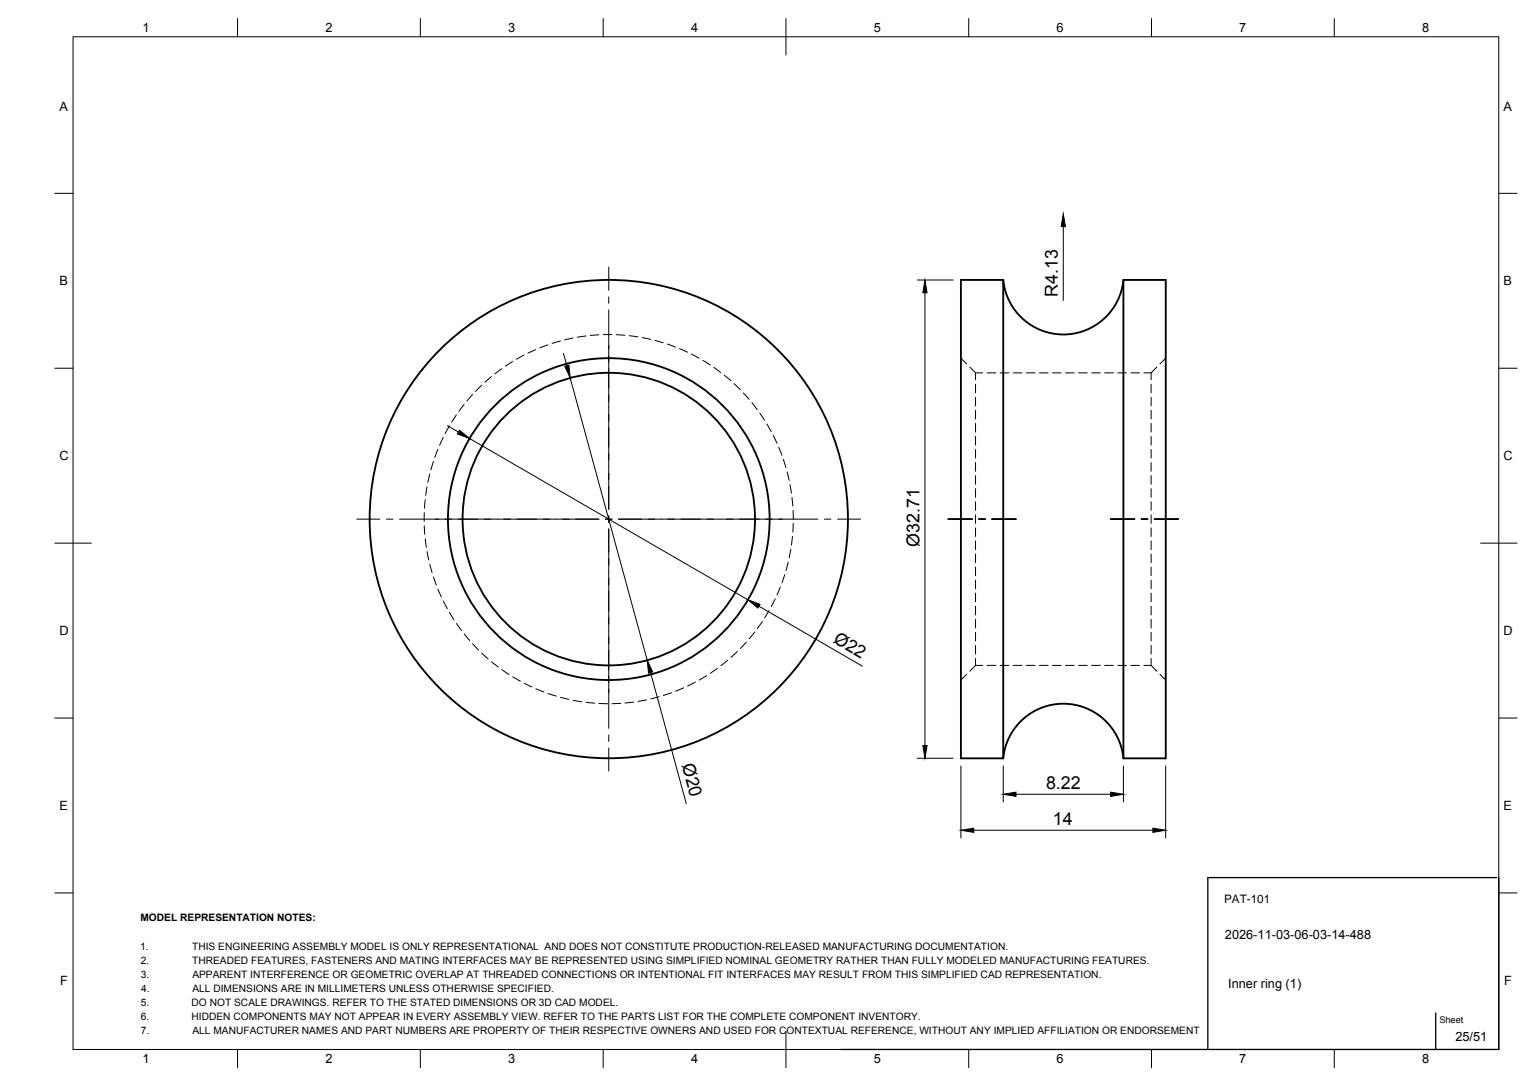
ISO-10303-21;
HEADER;
/* Generated by software containing ST-Developer
 * from STEP Tools, Inc. (www.steptools.com) 
 */

FILE_DESCRIPTION(
/* description */ ('Spur gear reduction stage 2-1 on bearing plates'),
/* implementation_level */ '2;1');

FILE_NAME(
/* name */ 'Inner ring (1).step',
/* time_stamp */ '2026-10-28T03:22:07-07:00',
/* author */ (''),
/* organization */ (''),
/* preprocessor_version */ 'ST-DEVELOPER v20.2',
/* originating_system */ 'Autodesk Translation Framework v15.17.0.0',
/* authorisation */ '');

FILE_SCHEMA (('AUTOMOTIVE_DESIGN { 1 0 10303 214 3 1 1 }'));
ENDSEC;

DATA;
#10=MECHANICAL_DESIGN_GEOMETRIC_PRESENTATION_REPRESENTATION('',(#972),#53909);
#827=TOROIDAL_SURFACE('',#12283,1.675,0.412776);
#844=CONICAL_SURFACE('',#12294,1.05,0.785398163397449);
#845=CONICAL_SURFACE('',#12301,1.05,0.785398163397449);
#879=SHAPE_REPRESENTATION_RELATIONSHIP('SRR','None',#54108,#922);
#922=ADVANCED_BREP_SHAPE_REPRESENTATION('',(#1028),#53882);
#972=STYLED_ITEM('',(#54397),#1028);
#1028=MANIFOLD_SOLID_BREP('Body1',#11298);
#1187=FACE_BOUND('',#2495,.T.);
#1188=FACE_BOUND('',#2498,.T.);
#1330=PLANE('',#12296);
#1331=PLANE('',#12299);
#1715=FACE_OUTER_BOUND('',#2490,.T.);
#1716=FACE_OUTER_BOUND('',#2491,.T.);
#1717=FACE_OUTER_BOUND('',#2492,.T.);
#1718=FACE_OUTER_BOUND('',#2493,.T.);
#1719=FACE_OUTER_BOUND('',#2494,.T.);
#1720=FACE_OUTER_BOUND('',#2496,.T.);
#1721=FACE_OUTER_BOUND('',#2497,.T.);
#1722=FACE_OUTER_BOUND('',#2499,.T.);
#2490=EDGE_LOOP('',(#8206,#8207,#8208,#8209,#8210,#8211));
#2491=EDGE_LOOP('',(#8212,#8213,#8214,#8215,#8216));
#2492=EDGE_LOOP('',(#8217,#8218,#8219,#8220));
#2493=EDGE_LOOP('',(#8221,#8222,#8223,#8224));
#2494=EDGE_LOOP('',(#8225));
#2495=EDGE_LOOP('',(#8226));
#2496=EDGE_LOOP('',(#8227,#8228,#8229,#8230,#8231));
#2497=EDGE_LOOP('',(#8232));
#2498=EDGE_LOOP('',(#8233));
#2499=EDGE_LOOP('',(#8234,#8235,#8236,#8237));
#3153=LINE('',#17238,#3794);
#3154=LINE('',#17244,#3795);
#3155=LINE('',#17248,#3796);
#3156=LINE('',#17254,#3797);
#3157=LINE('',#17259,#3798);
#3794=VECTOR('',#14126,1.63531);
#3795=VECTOR('',#14133,1.);
#3796=VECTOR('',#14138,1.05);
#3797=VECTOR('',#14147,1.63531);
#3798=VECTOR('',#14154,1.05);
#4496=CIRCLE('',#12284,1.63531);
#4497=CIRCLE('',#12285,1.63531);
#4498=CIRCLE('',#12286,0.412776);
#4499=CIRCLE('',#12287,1.63531);
#4500=CIRCLE('',#12288,1.63531);
#4501=CIRCLE('',#12290,1.63531);
#4502=CIRCLE('',#12292,1.);
#4503=CIRCLE('',#12293,1.);
#4504=CIRCLE('',#12295,1.1);
#4505=CIRCLE('',#12298,1.63531);
#4506=CIRCLE('',#12300,1.1);
#5074=VERTEX_POINT('',#17227);
#5075=VERTEX_POINT('',#17228);
#5076=VERTEX_POINT('',#17231);
#5077=VERTEX_POINT('',#17233);
#5078=VERTEX_POINT('',#17237);
#5079=VERTEX_POINT('',#17241);
#5080=VERTEX_POINT('',#17243);
#5081=VERTEX_POINT('',#17247);
#5082=VERTEX_POINT('',#17252);
#5083=VERTEX_POINT('',#17256);
#6245=EDGE_CURVE('',#5074,#5075,#4496,.T.);
#6246=EDGE_CURVE('',#5075,#5074,#4497,.T.);
#6247=EDGE_CURVE('',#5075,#5076,#4498,.T.);
#6248=EDGE_CURVE('',#5077,#5076,#4499,.T.);
#6249=EDGE_CURVE('',#5076,#5077,#4500,.T.);
#6250=EDGE_CURVE('',#5077,#5078,#3153,.T.);
#6251=EDGE_CURVE('',#5078,#5078,#4501,.T.);
#6252=EDGE_CURVE('',#5079,#5079,#4502,.T.);
#6253=EDGE_CURVE('',#5079,#5080,#3154,.T.);
#6254=EDGE_CURVE('',#5080,#5080,#4503,.T.);
#6255=EDGE_CURVE('',#5080,#5081,#3155,.T.);
#6256=EDGE_CURVE('',#5081,#5081,#4504,.T.);
#6257=EDGE_CURVE('',#5082,#5082,#4505,.T.);
#6258=EDGE_CURVE('',#5082,#5074,#3156,.T.);
#6259=EDGE_CURVE('',#5083,#5083,#4506,.T.);
#6260=EDGE_CURVE('',#5083,#5079,#3157,.T.);
#8206=ORIENTED_EDGE('',*,*,#6245,.F.);
#8207=ORIENTED_EDGE('',*,*,#6246,.F.);
#8208=ORIENTED_EDGE('',*,*,#6247,.T.);
#8209=ORIENTED_EDGE('',*,*,#6248,.F.);
#8210=ORIENTED_EDGE('',*,*,#6249,.F.);
#8211=ORIENTED_EDGE('',*,*,#6247,.F.);
#8212=ORIENTED_EDGE('',*,*,#6248,.T.);
#8213=ORIENTED_EDGE('',*,*,#6249,.T.);
#8214=ORIENTED_EDGE('',*,*,#6250,.T.);
#8215=ORIENTED_EDGE('',*,*,#6251,.T.);
#8216=ORIENTED_EDGE('',*,*,#6250,.F.);
#8217=ORIENTED_EDGE('',*,*,#6252,.T.);
#8218=ORIENTED_EDGE('',*,*,#6253,.T.);
#8219=ORIENTED_EDGE('',*,*,#6254,.F.);
#8220=ORIENTED_EDGE('',*,*,#6253,.F.);
#8221=ORIENTED_EDGE('',*,*,#6254,.T.);
#8222=ORIENTED_EDGE('',*,*,#6255,.T.);
#8223=ORIENTED_EDGE('',*,*,#6256,.F.);
#8224=ORIENTED_EDGE('',*,*,#6255,.F.);
#8225=ORIENTED_EDGE('',*,*,#6251,.F.);
#8226=ORIENTED_EDGE('',*,*,#6256,.T.);
#8227=ORIENTED_EDGE('',*,*,#6257,.F.);
#8228=ORIENTED_EDGE('',*,*,#6258,.T.);
#8229=ORIENTED_EDGE('',*,*,#6245,.T.);
#8230=ORIENTED_EDGE('',*,*,#6246,.T.);
#8231=ORIENTED_EDGE('',*,*,#6258,.F.);
#8232=ORIENTED_EDGE('',*,*,#6257,.T.);
#8233=ORIENTED_EDGE('',*,*,#6259,.F.);
#8234=ORIENTED_EDGE('',*,*,#6259,.T.);
#8235=ORIENTED_EDGE('',*,*,#6260,.T.);
#8236=ORIENTED_EDGE('',*,*,#6252,.F.);
#8237=ORIENTED_EDGE('',*,*,#6260,.F.);
#10512=CYLINDRICAL_SURFACE('',#12289,1.63531);
#10513=CYLINDRICAL_SURFACE('',#12291,1.);
#10514=CYLINDRICAL_SURFACE('',#12297,1.63531);
#10835=ADVANCED_FACE('',(#1715),#827,.F.);
#10836=ADVANCED_FACE('',(#1716),#10512,.T.);
#10837=ADVANCED_FACE('',(#1717),#10513,.F.);
#10838=ADVANCED_FACE('',(#1718),#844,.F.);
#10839=ADVANCED_FACE('',(#1719,#1187),#1330,.T.);
#10840=ADVANCED_FACE('',(#1720),#10514,.T.);
#10841=ADVANCED_FACE('',(#1721,#1188),#1331,.T.);
#10842=ADVANCED_FACE('',(#1722),#845,.F.);
#11298=CLOSED_SHELL('',(#10835,#10836,#10837,#10838,#10839,#10840,#10841,
#10842));
#12282=AXIS2_PLACEMENT_3D('',#17225,#14110,#14111);
#12283=AXIS2_PLACEMENT_3D('',#17226,#14112,#14113);
#12284=AXIS2_PLACEMENT_3D('',#17229,#14114,#14115);
#12285=AXIS2_PLACEMENT_3D('',#17230,#14116,#14117);
#12286=AXIS2_PLACEMENT_3D('',#17232,#14118,#14119);
#12287=AXIS2_PLACEMENT_3D('',#17234,#14120,#14121);
#12288=AXIS2_PLACEMENT_3D('',#17235,#14122,#14123);
#12289=AXIS2_PLACEMENT_3D('',#17236,#14124,#14125);
#12290=AXIS2_PLACEMENT_3D('',#17239,#14127,#14128);
#12291=AXIS2_PLACEMENT_3D('',#17240,#14129,#14130);
#12292=AXIS2_PLACEMENT_3D('',#17242,#14131,#14132);
#12293=AXIS2_PLACEMENT_3D('',#17245,#14134,#14135);
#12294=AXIS2_PLACEMENT_3D('',#17246,#14136,#14137);
#12295=AXIS2_PLACEMENT_3D('',#17249,#14139,#14140);
#12296=AXIS2_PLACEMENT_3D('',#17250,#14141,#14142);
#12297=AXIS2_PLACEMENT_3D('',#17251,#14143,#14144);
#12298=AXIS2_PLACEMENT_3D('',#17253,#14145,#14146);
#12299=AXIS2_PLACEMENT_3D('',#17255,#14148,#14149);
#12300=AXIS2_PLACEMENT_3D('',#17257,#14150,#14151);
#12301=AXIS2_PLACEMENT_3D('',#17258,#14152,#14153);
#14110=DIRECTION('axis',(0.,0.,1.));
#14111=DIRECTION('refdir',(1.,0.,0.));
#14112=DIRECTION('center_axis',(0.,-1.,0.));
#14113=DIRECTION('ref_axis',(0.,0.,-1.));
#14114=DIRECTION('center_axis',(0.,-1.,0.));
#14115=DIRECTION('ref_axis',(1.,0.,0.));
#14116=DIRECTION('center_axis',(0.,-1.,0.));
#14117=DIRECTION('ref_axis',(1.,0.,0.));
#14118=DIRECTION('center_axis',(1.,0.,1.22464679914735E-16));
#14119=DIRECTION('ref_axis',(-1.22464679914735E-16,0.,1.));
#14120=DIRECTION('center_axis',(0.,1.,0.));
#14121=DIRECTION('ref_axis',(1.,0.,0.));
#14122=DIRECTION('center_axis',(0.,1.,0.));
#14123=DIRECTION('ref_axis',(1.,0.,0.));
#14124=DIRECTION('center_axis',(0.,-1.,0.));
#14125=DIRECTION('ref_axis',(1.,0.,0.));
#14126=DIRECTION('',(0.,1.,0.));
#14127=DIRECTION('center_axis',(0.,-1.,0.));
#14128=DIRECTION('ref_axis',(1.,0.,0.));
#14129=DIRECTION('center_axis',(0.,-1.,0.));
#14130=DIRECTION('ref_axis',(1.,0.,0.));
#14131=DIRECTION('center_axis',(0.,-1.,0.));
#14132=DIRECTION('ref_axis',(1.,0.,0.));
#14133=DIRECTION('',(0.,1.,0.));
#14134=DIRECTION('center_axis',(0.,-1.,0.));
#14135=DIRECTION('ref_axis',(1.,0.,0.));
#14136=DIRECTION('center_axis',(0.,1.,0.));
#14137=DIRECTION('ref_axis',(1.,0.,0.));
#14138=DIRECTION('',(-0.707106781186548,0.707106781186547,-8.65956056235494E-17));
#14139=DIRECTION('center_axis',(0.,-1.,0.));
#14140=DIRECTION('ref_axis',(1.,0.,0.));
#14141=DIRECTION('center_axis',(0.,1.,0.));
#14142=DIRECTION('ref_axis',(0.,0.,1.));
#14143=DIRECTION('center_axis',(0.,-1.,0.));
#14144=DIRECTION('ref_axis',(1.,0.,0.));
#14145=DIRECTION('center_axis',(0.,-1.,0.));
#14146=DIRECTION('ref_axis',(1.,0.,0.));
#14147=DIRECTION('',(0.,1.,0.));
#14148=DIRECTION('center_axis',(0.,-1.,0.));
#14149=DIRECTION('ref_axis',(0.,0.,-1.));
#14150=DIRECTION('center_axis',(0.,-1.,0.));
#14151=DIRECTION('ref_axis',(1.,0.,0.));
#14152=DIRECTION('center_axis',(0.,-1.,0.));
#14153=DIRECTION('ref_axis',(1.,0.,0.));
#14154=DIRECTION('',(0.707106781186548,0.707106781186547,8.65956056235494E-17));
#17225=CARTESIAN_POINT('',(0.,0.,0.));
#17226=CARTESIAN_POINT('Origin',(0.,0.,0.));
#17227=CARTESIAN_POINT('',(-1.63531,-0.410863395882378,-2.00267715711366E-16));
#17228=CARTESIAN_POINT('',(-2.00267715711366E-16,-0.410863395882378,1.63531));
#17229=CARTESIAN_POINT('Origin',(0.,-0.410863395882378,0.));
#17230=CARTESIAN_POINT('Origin',(0.,-0.410863395882378,0.));
#17231=CARTESIAN_POINT('',(-2.00267715711366E-16,0.410863395882378,1.63531));
#17232=CARTESIAN_POINT('Origin',(-2.05128338857182E-16,0.,1.675));
#17233=CARTESIAN_POINT('',(-1.63531,0.410863395882378,2.00267715711366E-16));
#17234=CARTESIAN_POINT('Origin',(0.,0.410863395882378,0.));
#17235=CARTESIAN_POINT('Origin',(0.,0.410863395882378,0.));
#17236=CARTESIAN_POINT('Origin',(0.,0.,0.));
#17237=CARTESIAN_POINT('',(-1.63531,0.7,-2.00267715711366E-16));
#17238=CARTESIAN_POINT('',(-1.63531,0.,-2.00267715711366E-16));
#17239=CARTESIAN_POINT('Origin',(0.,0.7,0.));
#17240=CARTESIAN_POINT('Origin',(0.,0.,0.));
#17241=CARTESIAN_POINT('',(-1.,-0.6,-1.22464679914735E-16));
#17242=CARTESIAN_POINT('Origin',(0.,-0.6,0.));
#17243=CARTESIAN_POINT('',(-1.,0.6,-1.22464679914735E-16));
#17244=CARTESIAN_POINT('',(-1.,0.,-1.22464679914735E-16));
#17245=CARTESIAN_POINT('Origin',(0.,0.6,0.));
#17246=CARTESIAN_POINT('Origin',(0.,0.65,0.));
#17247=CARTESIAN_POINT('',(-1.1,0.7,-1.34711147906209E-16));
#17248=CARTESIAN_POINT('',(-1.05,0.65,-1.28587913910472E-16));
#17249=CARTESIAN_POINT('Origin',(0.,0.7,0.));
#17250=CARTESIAN_POINT('Origin',(1.63531,0.7,0.));
#17251=CARTESIAN_POINT('Origin',(0.,0.,0.));
#17252=CARTESIAN_POINT('',(-1.63531,-0.7,-2.00267715711366E-16));
#17253=CARTESIAN_POINT('Origin',(0.,-0.7,0.));
#17254=CARTESIAN_POINT('',(-1.63531,0.,-2.00267715711366E-16));
#17255=CARTESIAN_POINT('Origin',(1.1,-0.7,0.));
#17256=CARTESIAN_POINT('',(-1.1,-0.7,-1.34711147906209E-16));
#17257=CARTESIAN_POINT('Origin',(0.,-0.7,0.));
#17258=CARTESIAN_POINT('Origin',(0.,-0.65,0.));
#17259=CARTESIAN_POINT('',(-1.05,-0.65,-1.28587913910472E-16));
#53832=UNCERTAINTY_MEASURE_WITH_UNIT(LENGTH_MEASURE(0.001),#53910,
'DISTANCE_ACCURACY_VALUE',
'Maximum model space distance between geometric entities at asserted c
onnectivities');
#53859=UNCERTAINTY_MEASURE_WITH_UNIT(LENGTH_MEASURE(0.001),#53910,
'DISTANCE_ACCURACY_VALUE',
'Maximum model space distance between geometric entities at asserted c
onnectivities');
#53882=(
GEOMETRIC_REPRESENTATION_CONTEXT(3)
GLOBAL_UNCERTAINTY_ASSIGNED_CONTEXT((#53832))
GLOBAL_UNIT_ASSIGNED_CONTEXT((#53910,#53912,#53913))
REPRESENTATION_CONTEXT('','3D')
);
#53909=(
GEOMETRIC_REPRESENTATION_CONTEXT(3)
GLOBAL_UNCERTAINTY_ASSIGNED_CONTEXT((#53859))
GLOBAL_UNIT_ASSIGNED_CONTEXT((#53910,#53912,#53913))
REPRESENTATION_CONTEXT('','3D')
);
#53910=(
LENGTH_UNIT()
NAMED_UNIT(*)
SI_UNIT(.CENTI.,.METRE.)
);
#53912=(
NAMED_UNIT(*)
PLANE_ANGLE_UNIT()
SI_UNIT($,.RADIAN.)
);
#53913=(
NAMED_UNIT(*)
SI_UNIT($,.STERADIAN.)
SOLID_ANGLE_UNIT()
);
#53936=SHAPE_DEFINITION_REPRESENTATION(#53990,#54108);
#53990=PRODUCT_DEFINITION_SHAPE('',$,#54158);
#54108=SHAPE_REPRESENTATION('',(#12282),#53882);
#54135=PRODUCT_DEFINITION_CONTEXT('part definition',#54284,'design');
#54158=PRODUCT_DEFINITION('Inner ring (1)','Inner ring (1)',#54207,#54135);
#54207=PRODUCT_DEFINITION_FORMATION('',$,#54308);
#54284=APPLICATION_CONTEXT(
'Core Data for Automotive Mechanical Design Process');
#54285=PRODUCT_CONTEXT('part definition',#54284,'mechanical');
#54308=PRODUCT('Inner ring (1)','Inner ring (1)','Inner ring (1)',(#54285));
#54391=COLOUR_RGB('Grey',0.48,0.52,0.57);
#54392=FILL_AREA_STYLE_COLOUR('',#54391);
#54393=FILL_AREA_STYLE('',(#54392));
#54394=SURFACE_STYLE_FILL_AREA(#54393);
#54395=SURFACE_SIDE_STYLE('',(#54394));
#54396=SURFACE_STYLE_USAGE(.BOTH.,#54395);
#54397=PRESENTATION_STYLE_ASSIGNMENT((#54396));
ENDSEC;
END-ISO-10303-21;
